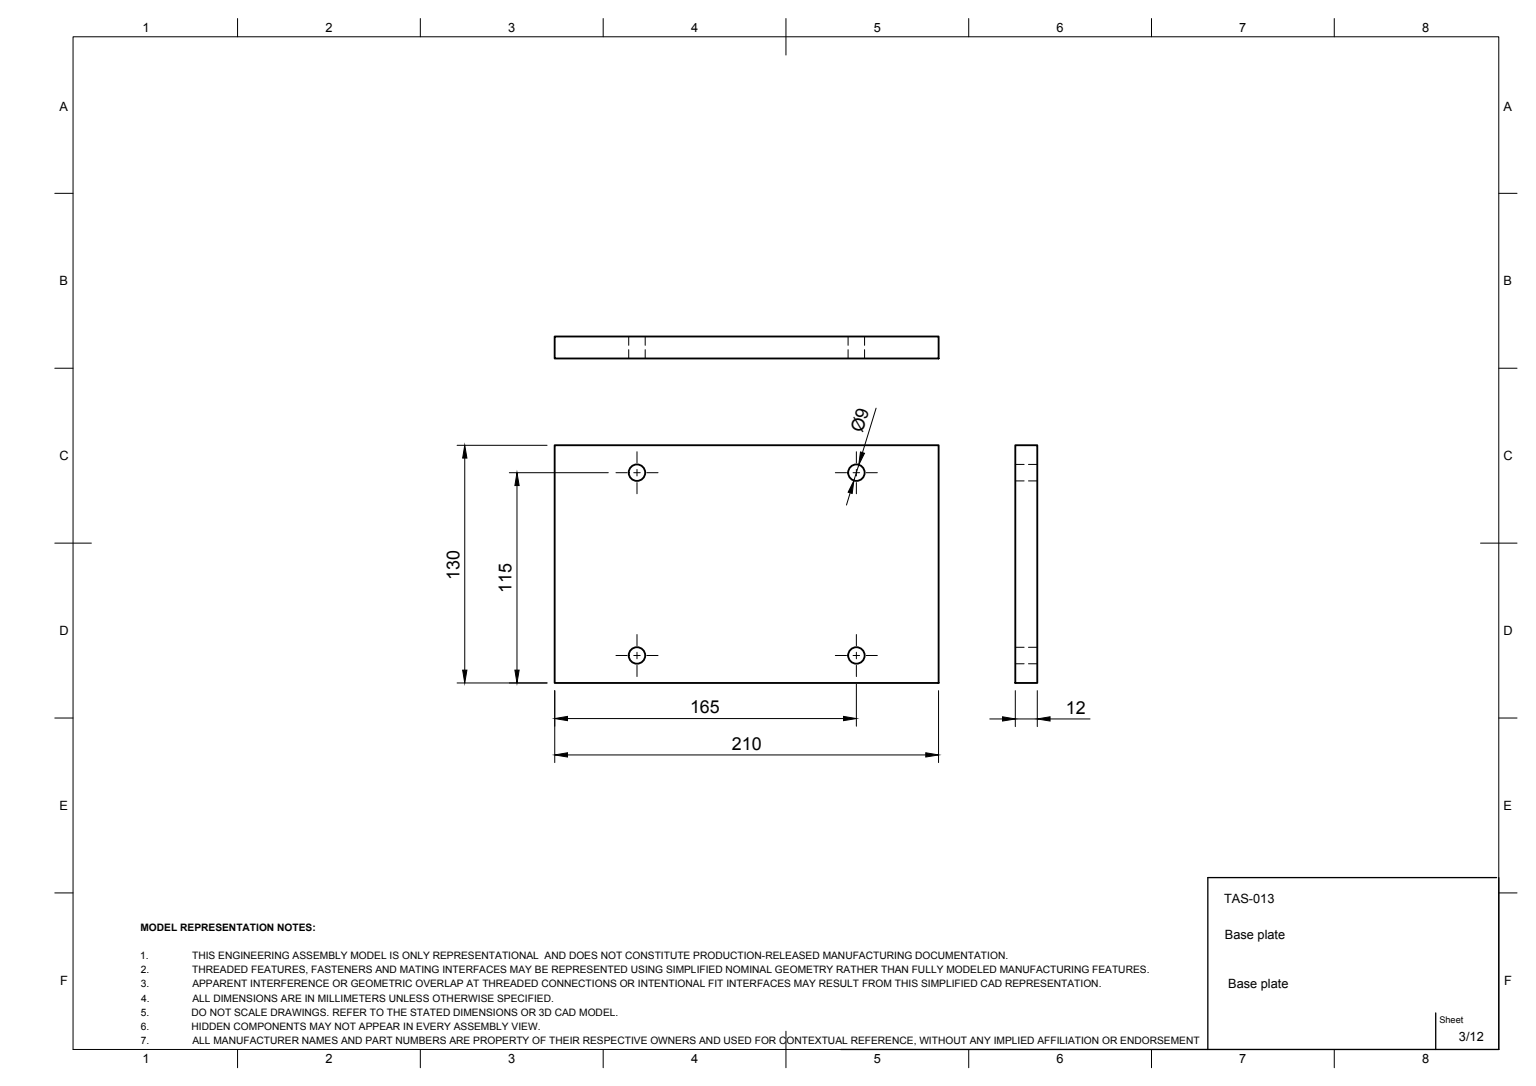
ISO-10303-21;
HEADER;
/* Generated by software containing ST-Developer
 * from STEP Tools, Inc. (www.steptools.com) 
 */

FILE_DESCRIPTION(
/* description */ (
'Independent guided parallel-jaw bracket clamp. Two12mm guide rods, re
placeable bronze sleeves, captured swiveling spindle, replaceable jaw 
pads and modeled M16x2 screw. Native slider/revolute joints linked2mm 
per revolution. Nominal opening0..122 with initial28mm. Base and two i
dentical supports welded. Standard fits, weld details and clamp load r
equire engineering selection.'),
/* implementation_level */ '2;1');

FILE_NAME(
/* name */ 'Base plate.step',
/* time_stamp */ '2026-11-14T09:15:44-08:00',
/* author */ (''),
/* organization */ (''),
/* preprocessor_version */ 'ST-DEVELOPER v20.2',
/* originating_system */ 'Autodesk Translation Framework v15.17.0.0',
/* authorisation */ '');

FILE_SCHEMA (('AUTOMOTIVE_DESIGN { 1 0 10303 214 3 1 1 }'));
ENDSEC;

DATA;
#10=MECHANICAL_DESIGN_GEOMETRIC_PRESENTATION_REPRESENTATION('',(#915),#105806);
#891=SHAPE_REPRESENTATION_RELATIONSHIP('SRR','None',#105859,#903);
#903=ADVANCED_BREP_SHAPE_REPRESENTATION('',(#927),#105794);
#915=STYLED_ITEM('',(#105928),#927);
#927=MANIFOLD_SOLID_BREP('Body1',#7202);
#939=FACE_BOUND('',#1346,.T.);
#940=FACE_BOUND('',#1347,.T.);
#941=FACE_BOUND('',#1348,.T.);
#942=FACE_BOUND('',#1349,.T.);
#943=FACE_BOUND('',#1351,.T.);
#944=FACE_BOUND('',#1352,.T.);
#945=FACE_BOUND('',#1353,.T.);
#946=FACE_BOUND('',#1354,.T.);
#998=PLANE('',#7361);
#999=PLANE('',#7362);
#1000=PLANE('',#7363);
#1001=PLANE('',#7364);
#1002=PLANE('',#7365);
#1003=PLANE('',#7366);
#1065=FACE_OUTER_BOUND('',#1337,.T.);
#1066=FACE_OUTER_BOUND('',#1338,.T.);
#1067=FACE_OUTER_BOUND('',#1339,.T.);
#1068=FACE_OUTER_BOUND('',#1340,.T.);
#1069=FACE_OUTER_BOUND('',#1341,.T.);
#1070=FACE_OUTER_BOUND('',#1342,.T.);
#1071=FACE_OUTER_BOUND('',#1343,.T.);
#1072=FACE_OUTER_BOUND('',#1344,.T.);
#1073=FACE_OUTER_BOUND('',#1345,.T.);
#1074=FACE_OUTER_BOUND('',#1350,.T.);
#1337=EDGE_LOOP('',(#4413,#4414,#4415,#4416));
#1338=EDGE_LOOP('',(#4417,#4418,#4419,#4420));
#1339=EDGE_LOOP('',(#4421,#4422,#4423,#4424));
#1340=EDGE_LOOP('',(#4425,#4426,#4427,#4428));
#1341=EDGE_LOOP('',(#4429,#4430,#4431,#4432));
#1342=EDGE_LOOP('',(#4433,#4434,#4435,#4436));
#1343=EDGE_LOOP('',(#4437,#4438,#4439,#4440));
#1344=EDGE_LOOP('',(#4441,#4442,#4443,#4444));
#1345=EDGE_LOOP('',(#4445,#4446,#4447,#4448));
#1346=EDGE_LOOP('',(#4449));
#1347=EDGE_LOOP('',(#4450));
#1348=EDGE_LOOP('',(#4451));
#1349=EDGE_LOOP('',(#4452));
#1350=EDGE_LOOP('',(#4453,#4454,#4455,#4456));
#1351=EDGE_LOOP('',(#4457));
#1352=EDGE_LOOP('',(#4458));
#1353=EDGE_LOOP('',(#4459));
#1354=EDGE_LOOP('',(#4460));
#1668=LINE('',#8821,#1948);
#1669=LINE('',#8827,#1949);
#1670=LINE('',#8833,#1950);
#1671=LINE('',#8839,#1951);
#1672=LINE('',#8844,#1952);
#1673=LINE('',#8846,#1953);
#1674=LINE('',#8848,#1954);
#1675=LINE('',#8849,#1955);
#1676=LINE('',#8852,#1956);
#1677=LINE('',#8854,#1957);
#1678=LINE('',#8855,#1958);
#1679=LINE('',#8858,#1959);
#1680=LINE('',#8860,#1960);
#1681=LINE('',#8861,#1961);
#1682=LINE('',#8863,#1962);
#1683=LINE('',#8864,#1963);
#1948=VECTOR('',#7751,4.5);
#1949=VECTOR('',#7758,4.5);
#1950=VECTOR('',#7765,4.5);
#1951=VECTOR('',#7772,4.5);
#1952=VECTOR('',#7777,10.);
#1953=VECTOR('',#7778,10.);
#1954=VECTOR('',#7779,10.);
#1955=VECTOR('',#7780,10.);
#1956=VECTOR('',#7783,10.);
#1957=VECTOR('',#7784,10.);
#1958=VECTOR('',#7785,10.);
#1959=VECTOR('',#7788,10.);
#1960=VECTOR('',#7789,10.);
#1961=VECTOR('',#7790,10.);
#1962=VECTOR('',#7793,10.);
#1963=VECTOR('',#7794,10.);
#2228=CIRCLE('',#7350,4.5);
#2229=CIRCLE('',#7351,4.5);
#2230=CIRCLE('',#7353,4.5);
#2231=CIRCLE('',#7354,4.5);
#2232=CIRCLE('',#7356,4.5);
#2233=CIRCLE('',#7357,4.5);
#2234=CIRCLE('',#7359,4.5);
#2235=CIRCLE('',#7360,4.5);
#2326=VERTEX_POINT('',#8818);
#2327=VERTEX_POINT('',#8820);
#2328=VERTEX_POINT('',#8824);
#2329=VERTEX_POINT('',#8826);
#2330=VERTEX_POINT('',#8830);
#2331=VERTEX_POINT('',#8832);
#2332=VERTEX_POINT('',#8836);
#2333=VERTEX_POINT('',#8838);
#2334=VERTEX_POINT('',#8842);
#2335=VERTEX_POINT('',#8843);
#2336=VERTEX_POINT('',#8845);
#2337=VERTEX_POINT('',#8847);
#2338=VERTEX_POINT('',#8851);
#2339=VERTEX_POINT('',#8853);
#2340=VERTEX_POINT('',#8857);
#2341=VERTEX_POINT('',#8859);
#3251=EDGE_CURVE('',#2326,#2326,#2228,.T.);
#3252=EDGE_CURVE('',#2326,#2327,#1668,.T.);
#3253=EDGE_CURVE('',#2327,#2327,#2229,.T.);
#3254=EDGE_CURVE('',#2328,#2328,#2230,.T.);
#3255=EDGE_CURVE('',#2328,#2329,#1669,.T.);
#3256=EDGE_CURVE('',#2329,#2329,#2231,.T.);
#3257=EDGE_CURVE('',#2330,#2330,#2232,.T.);
#3258=EDGE_CURVE('',#2330,#2331,#1670,.T.);
#3259=EDGE_CURVE('',#2331,#2331,#2233,.T.);
#3260=EDGE_CURVE('',#2332,#2332,#2234,.T.);
#3261=EDGE_CURVE('',#2332,#2333,#1671,.T.);
#3262=EDGE_CURVE('',#2333,#2333,#2235,.T.);
#3263=EDGE_CURVE('',#2334,#2335,#1672,.F.);
#3264=EDGE_CURVE('',#2335,#2336,#1673,.T.);
#3265=EDGE_CURVE('',#2337,#2336,#1674,.F.);
#3266=EDGE_CURVE('',#2334,#2337,#1675,.F.);
#3267=EDGE_CURVE('',#2338,#2334,#1676,.F.);
#3268=EDGE_CURVE('',#2339,#2337,#1677,.F.);
#3269=EDGE_CURVE('',#2338,#2339,#1678,.F.);
#3270=EDGE_CURVE('',#2340,#2338,#1679,.F.);
#3271=EDGE_CURVE('',#2341,#2339,#1680,.F.);
#3272=EDGE_CURVE('',#2340,#2341,#1681,.T.);
#3273=EDGE_CURVE('',#2335,#2340,#1682,.F.);
#3274=EDGE_CURVE('',#2336,#2341,#1683,.F.);
#4413=ORIENTED_EDGE('',*,*,#3251,.F.);
#4414=ORIENTED_EDGE('',*,*,#3252,.T.);
#4415=ORIENTED_EDGE('',*,*,#3253,.F.);
#4416=ORIENTED_EDGE('',*,*,#3252,.F.);
#4417=ORIENTED_EDGE('',*,*,#3254,.F.);
#4418=ORIENTED_EDGE('',*,*,#3255,.T.);
#4419=ORIENTED_EDGE('',*,*,#3256,.F.);
#4420=ORIENTED_EDGE('',*,*,#3255,.F.);
#4421=ORIENTED_EDGE('',*,*,#3257,.F.);
#4422=ORIENTED_EDGE('',*,*,#3258,.T.);
#4423=ORIENTED_EDGE('',*,*,#3259,.F.);
#4424=ORIENTED_EDGE('',*,*,#3258,.F.);
#4425=ORIENTED_EDGE('',*,*,#3260,.F.);
#4426=ORIENTED_EDGE('',*,*,#3261,.T.);
#4427=ORIENTED_EDGE('',*,*,#3262,.F.);
#4428=ORIENTED_EDGE('',*,*,#3261,.F.);
#4429=ORIENTED_EDGE('',*,*,#3263,.T.);
#4430=ORIENTED_EDGE('',*,*,#3264,.T.);
#4431=ORIENTED_EDGE('',*,*,#3265,.F.);
#4432=ORIENTED_EDGE('',*,*,#3266,.F.);
#4433=ORIENTED_EDGE('',*,*,#3267,.T.);
#4434=ORIENTED_EDGE('',*,*,#3266,.T.);
#4435=ORIENTED_EDGE('',*,*,#3268,.F.);
#4436=ORIENTED_EDGE('',*,*,#3269,.F.);
#4437=ORIENTED_EDGE('',*,*,#3270,.T.);
#4438=ORIENTED_EDGE('',*,*,#3269,.T.);
#4439=ORIENTED_EDGE('',*,*,#3271,.F.);
#4440=ORIENTED_EDGE('',*,*,#3272,.F.);
#4441=ORIENTED_EDGE('',*,*,#3273,.T.);
#4442=ORIENTED_EDGE('',*,*,#3272,.T.);
#4443=ORIENTED_EDGE('',*,*,#3274,.F.);
#4444=ORIENTED_EDGE('',*,*,#3264,.F.);
#4445=ORIENTED_EDGE('',*,*,#3274,.T.);
#4446=ORIENTED_EDGE('',*,*,#3271,.T.);
#4447=ORIENTED_EDGE('',*,*,#3268,.T.);
#4448=ORIENTED_EDGE('',*,*,#3265,.T.);
#4449=ORIENTED_EDGE('',*,*,#3251,.T.);
#4450=ORIENTED_EDGE('',*,*,#3254,.T.);
#4451=ORIENTED_EDGE('',*,*,#3257,.T.);
#4452=ORIENTED_EDGE('',*,*,#3260,.T.);
#4453=ORIENTED_EDGE('',*,*,#3273,.F.);
#4454=ORIENTED_EDGE('',*,*,#3263,.F.);
#4455=ORIENTED_EDGE('',*,*,#3267,.F.);
#4456=ORIENTED_EDGE('',*,*,#3270,.F.);
#4457=ORIENTED_EDGE('',*,*,#3253,.T.);
#4458=ORIENTED_EDGE('',*,*,#3256,.T.);
#4459=ORIENTED_EDGE('',*,*,#3259,.T.);
#4460=ORIENTED_EDGE('',*,*,#3262,.T.);
#6737=CYLINDRICAL_SURFACE('',#7349,4.5);
#6738=CYLINDRICAL_SURFACE('',#7352,4.5);
#6739=CYLINDRICAL_SURFACE('',#7355,4.5);
#6740=CYLINDRICAL_SURFACE('',#7358,4.5);
#6930=ADVANCED_FACE('',(#1065),#6737,.F.);
#6931=ADVANCED_FACE('',(#1066),#6738,.F.);
#6932=ADVANCED_FACE('',(#1067),#6739,.F.);
#6933=ADVANCED_FACE('',(#1068),#6740,.F.);
#6934=ADVANCED_FACE('',(#1069),#998,.T.);
#6935=ADVANCED_FACE('',(#1070),#999,.T.);
#6936=ADVANCED_FACE('',(#1071),#1000,.T.);
#6937=ADVANCED_FACE('',(#1072),#1001,.T.);
#6938=ADVANCED_FACE('',(#1073,#939,#940,#941,#942),#1002,.T.);
#6939=ADVANCED_FACE('',(#1074,#943,#944,#945,#946),#1003,.F.);
#7202=CLOSED_SHELL('',(#6930,#6931,#6932,#6933,#6934,#6935,#6936,#6937,
#6938,#6939));
#7348=AXIS2_PLACEMENT_3D('',#8816,#7745,#7746);
#7349=AXIS2_PLACEMENT_3D('',#8817,#7747,#7748);
#7350=AXIS2_PLACEMENT_3D('',#8819,#7749,#7750);
#7351=AXIS2_PLACEMENT_3D('',#8822,#7752,#7753);
#7352=AXIS2_PLACEMENT_3D('',#8823,#7754,#7755);
#7353=AXIS2_PLACEMENT_3D('',#8825,#7756,#7757);
#7354=AXIS2_PLACEMENT_3D('',#8828,#7759,#7760);
#7355=AXIS2_PLACEMENT_3D('',#8829,#7761,#7762);
#7356=AXIS2_PLACEMENT_3D('',#8831,#7763,#7764);
#7357=AXIS2_PLACEMENT_3D('',#8834,#7766,#7767);
#7358=AXIS2_PLACEMENT_3D('',#8835,#7768,#7769);
#7359=AXIS2_PLACEMENT_3D('',#8837,#7770,#7771);
#7360=AXIS2_PLACEMENT_3D('',#8840,#7773,#7774);
#7361=AXIS2_PLACEMENT_3D('',#8841,#7775,#7776);
#7362=AXIS2_PLACEMENT_3D('',#8850,#7781,#7782);
#7363=AXIS2_PLACEMENT_3D('',#8856,#7786,#7787);
#7364=AXIS2_PLACEMENT_3D('',#8862,#7791,#7792);
#7365=AXIS2_PLACEMENT_3D('',#8865,#7795,#7796);
#7366=AXIS2_PLACEMENT_3D('',#8866,#7797,#7798);
#7745=DIRECTION('axis',(0.,0.,1.));
#7746=DIRECTION('refdir',(1.,0.,0.));
#7747=DIRECTION('center_axis',(0.,0.,-1.));
#7748=DIRECTION('ref_axis',(1.,0.,0.));
#7749=DIRECTION('center_axis',(0.,0.,-1.));
#7750=DIRECTION('ref_axis',(1.,0.,0.));
#7751=DIRECTION('',(0.,0.,-1.));
#7752=DIRECTION('center_axis',(0.,0.,1.));
#7753=DIRECTION('ref_axis',(1.,0.,0.));
#7754=DIRECTION('center_axis',(0.,0.,-1.));
#7755=DIRECTION('ref_axis',(1.,0.,0.));
#7756=DIRECTION('center_axis',(0.,0.,-1.));
#7757=DIRECTION('ref_axis',(1.,0.,0.));
#7758=DIRECTION('',(0.,0.,-1.));
#7759=DIRECTION('center_axis',(0.,0.,1.));
#7760=DIRECTION('ref_axis',(1.,0.,0.));
#7761=DIRECTION('center_axis',(0.,0.,-1.));
#7762=DIRECTION('ref_axis',(1.,0.,0.));
#7763=DIRECTION('center_axis',(0.,0.,-1.));
#7764=DIRECTION('ref_axis',(1.,0.,0.));
#7765=DIRECTION('',(0.,0.,-1.));
#7766=DIRECTION('center_axis',(0.,0.,1.));
#7767=DIRECTION('ref_axis',(1.,0.,0.));
#7768=DIRECTION('center_axis',(0.,0.,-1.));
#7769=DIRECTION('ref_axis',(1.,0.,0.));
#7770=DIRECTION('center_axis',(0.,0.,-1.));
#7771=DIRECTION('ref_axis',(1.,0.,0.));
#7772=DIRECTION('',(0.,0.,-1.));
#7773=DIRECTION('center_axis',(0.,0.,1.));
#7774=DIRECTION('ref_axis',(1.,0.,0.));
#7775=DIRECTION('center_axis',(0.,1.,0.));
#7776=DIRECTION('ref_axis',(-1.,0.,0.));
#7777=DIRECTION('',(1.,0.,0.));
#7778=DIRECTION('',(0.,0.,1.));
#7779=DIRECTION('',(1.,0.,0.));
#7780=DIRECTION('',(0.,0.,-1.));
#7781=DIRECTION('center_axis',(1.,0.,0.));
#7782=DIRECTION('ref_axis',(0.,1.,0.));
#7783=DIRECTION('',(0.,-1.,0.));
#7784=DIRECTION('',(0.,-1.,0.));
#7785=DIRECTION('',(0.,0.,-1.));
#7786=DIRECTION('center_axis',(0.,-1.,0.));
#7787=DIRECTION('ref_axis',(1.,0.,0.));
#7788=DIRECTION('',(-1.,0.,0.));
#7789=DIRECTION('',(-1.,0.,0.));
#7790=DIRECTION('',(0.,0.,1.));
#7791=DIRECTION('center_axis',(-1.,0.,0.));
#7792=DIRECTION('ref_axis',(0.,-1.,0.));
#7793=DIRECTION('',(0.,1.,0.));
#7794=DIRECTION('',(0.,1.,0.));
#7795=DIRECTION('center_axis',(0.,0.,1.));
#7796=DIRECTION('ref_axis',(1.,0.,0.));
#7797=DIRECTION('center_axis',(0.,0.,1.));
#7798=DIRECTION('ref_axis',(1.,0.,0.));
#8816=CARTESIAN_POINT('',(0.,0.,0.));
#8817=CARTESIAN_POINT('Origin',(160.,-50.,6.));
#8818=CARTESIAN_POINT('',(155.5,-50.,12.));
#8819=CARTESIAN_POINT('Origin',(160.,-50.,12.));
#8820=CARTESIAN_POINT('',(155.5,-50.,0.));
#8821=CARTESIAN_POINT('',(155.5,-50.,6.));
#8822=CARTESIAN_POINT('Origin',(160.,-50.,0.));
#8823=CARTESIAN_POINT('Origin',(40.,-50.,6.));
#8824=CARTESIAN_POINT('',(35.5,-50.,12.));
#8825=CARTESIAN_POINT('Origin',(40.,-50.,12.));
#8826=CARTESIAN_POINT('',(35.5,-50.,0.));
#8827=CARTESIAN_POINT('',(35.5,-50.,6.));
#8828=CARTESIAN_POINT('Origin',(40.,-50.,0.));
#8829=CARTESIAN_POINT('Origin',(40.,50.,6.));
#8830=CARTESIAN_POINT('',(35.5,50.,12.));
#8831=CARTESIAN_POINT('Origin',(40.,50.,12.));
#8832=CARTESIAN_POINT('',(35.5,50.,0.));
#8833=CARTESIAN_POINT('',(35.5,50.,6.));
#8834=CARTESIAN_POINT('Origin',(40.,50.,0.));
#8835=CARTESIAN_POINT('Origin',(160.,50.,6.));
#8836=CARTESIAN_POINT('',(155.5,50.,12.));
#8837=CARTESIAN_POINT('Origin',(160.,50.,12.));
#8838=CARTESIAN_POINT('',(155.5,50.,0.));
#8839=CARTESIAN_POINT('',(155.5,50.,6.));
#8840=CARTESIAN_POINT('Origin',(160.,50.,0.));
#8841=CARTESIAN_POINT('Origin',(200.,65.,0.));
#8842=CARTESIAN_POINT('',(205.,65.,0.));
#8843=CARTESIAN_POINT('',(-5.,65.,0.));
#8844=CARTESIAN_POINT('',(150.,65.,0.));
#8845=CARTESIAN_POINT('',(-5.,65.,12.));
#8846=CARTESIAN_POINT('',(-5.,65.,0.));
#8847=CARTESIAN_POINT('',(205.,65.,12.));
#8848=CARTESIAN_POINT('',(150.,65.,12.));
#8849=CARTESIAN_POINT('',(205.,65.,0.));
#8850=CARTESIAN_POINT('Origin',(205.,-60.,0.));
#8851=CARTESIAN_POINT('',(205.,-65.,0.));
#8852=CARTESIAN_POINT('',(205.,-30.,0.));
#8853=CARTESIAN_POINT('',(205.,-65.,12.));
#8854=CARTESIAN_POINT('',(205.,-30.,12.));
#8855=CARTESIAN_POINT('',(205.,-65.,0.));
#8856=CARTESIAN_POINT('Origin',(0.,-65.,0.));
#8857=CARTESIAN_POINT('',(-5.,-65.,0.));
#8858=CARTESIAN_POINT('',(50.,-65.,0.));
#8859=CARTESIAN_POINT('',(-5.,-65.,12.));
#8860=CARTESIAN_POINT('',(50.,-65.,12.));
#8861=CARTESIAN_POINT('',(-5.,-65.,0.));
#8862=CARTESIAN_POINT('Origin',(-5.,60.,0.));
#8863=CARTESIAN_POINT('',(-5.,30.,0.));
#8864=CARTESIAN_POINT('',(-5.,30.,12.));
#8865=CARTESIAN_POINT('Origin',(100.,0.,12.));
#8866=CARTESIAN_POINT('Origin',(100.,0.,0.));
#105780=UNCERTAINTY_MEASURE_WITH_UNIT(LENGTH_MEASURE(0.01),#105807,
'DISTANCE_ACCURACY_VALUE',
'Maximum model space distance between geometric entities at asserted c
onnectivities');
#105792=UNCERTAINTY_MEASURE_WITH_UNIT(LENGTH_MEASURE(0.01),#105807,
'DISTANCE_ACCURACY_VALUE',
'Maximum model space distance between geometric entities at asserted c
onnectivities');
#105794=(
GEOMETRIC_REPRESENTATION_CONTEXT(3)
GLOBAL_UNCERTAINTY_ASSIGNED_CONTEXT((#105780))
GLOBAL_UNIT_ASSIGNED_CONTEXT((#105807,#105809,#105810))
REPRESENTATION_CONTEXT('','3D')
);
#105806=(
GEOMETRIC_REPRESENTATION_CONTEXT(3)
GLOBAL_UNCERTAINTY_ASSIGNED_CONTEXT((#105792))
GLOBAL_UNIT_ASSIGNED_CONTEXT((#105807,#105809,#105810))
REPRESENTATION_CONTEXT('','3D')
);
#105807=(
LENGTH_UNIT()
NAMED_UNIT(*)
SI_UNIT(.MILLI.,.METRE.)
);
#105809=(
NAMED_UNIT(*)
PLANE_ANGLE_UNIT()
SI_UNIT($,.RADIAN.)
);
#105810=(
NAMED_UNIT(*)
SI_UNIT($,.STERADIAN.)
SOLID_ANGLE_UNIT()
);
#105812=SHAPE_DEFINITION_REPRESENTATION(#105825,#105859);
#105825=PRODUCT_DEFINITION_SHAPE('',$,#105873);
#105859=SHAPE_REPRESENTATION('',(#7348),#105794);
#105871=PRODUCT_DEFINITION_CONTEXT('part definition',#105912,'design');
#105873=PRODUCT_DEFINITION('Base plate','Base plate',#105886,#105871);
#105886=PRODUCT_DEFINITION_FORMATION('',$,#105915);
#105912=APPLICATION_CONTEXT(
'Core Data for Automotive Mechanical Design Process');
#105913=PRODUCT_CONTEXT('part definition',#105912,'mechanical');
#105915=PRODUCT('Base plate','Base plate','Base plate',(#105913));
#105928=PRESENTATION_STYLE_ASSIGNMENT((#105934));
#105934=SURFACE_STYLE_USAGE(.BOTH.,#105940);
#105940=SURFACE_SIDE_STYLE('',(#105946));
#105946=SURFACE_STYLE_FILL_AREA(#105952);
#105952=FILL_AREA_STYLE('Opaque(104,114,127)',(#105958));
#105958=FILL_AREA_STYLE_COLOUR('Opaque(104,114,127)',#105964);
#105964=COLOUR_RGB('Opaque(104,114,127)',0.407843137254902,0.447058823529412,
0.498039215686275);
ENDSEC;
END-ISO-10303-21;
